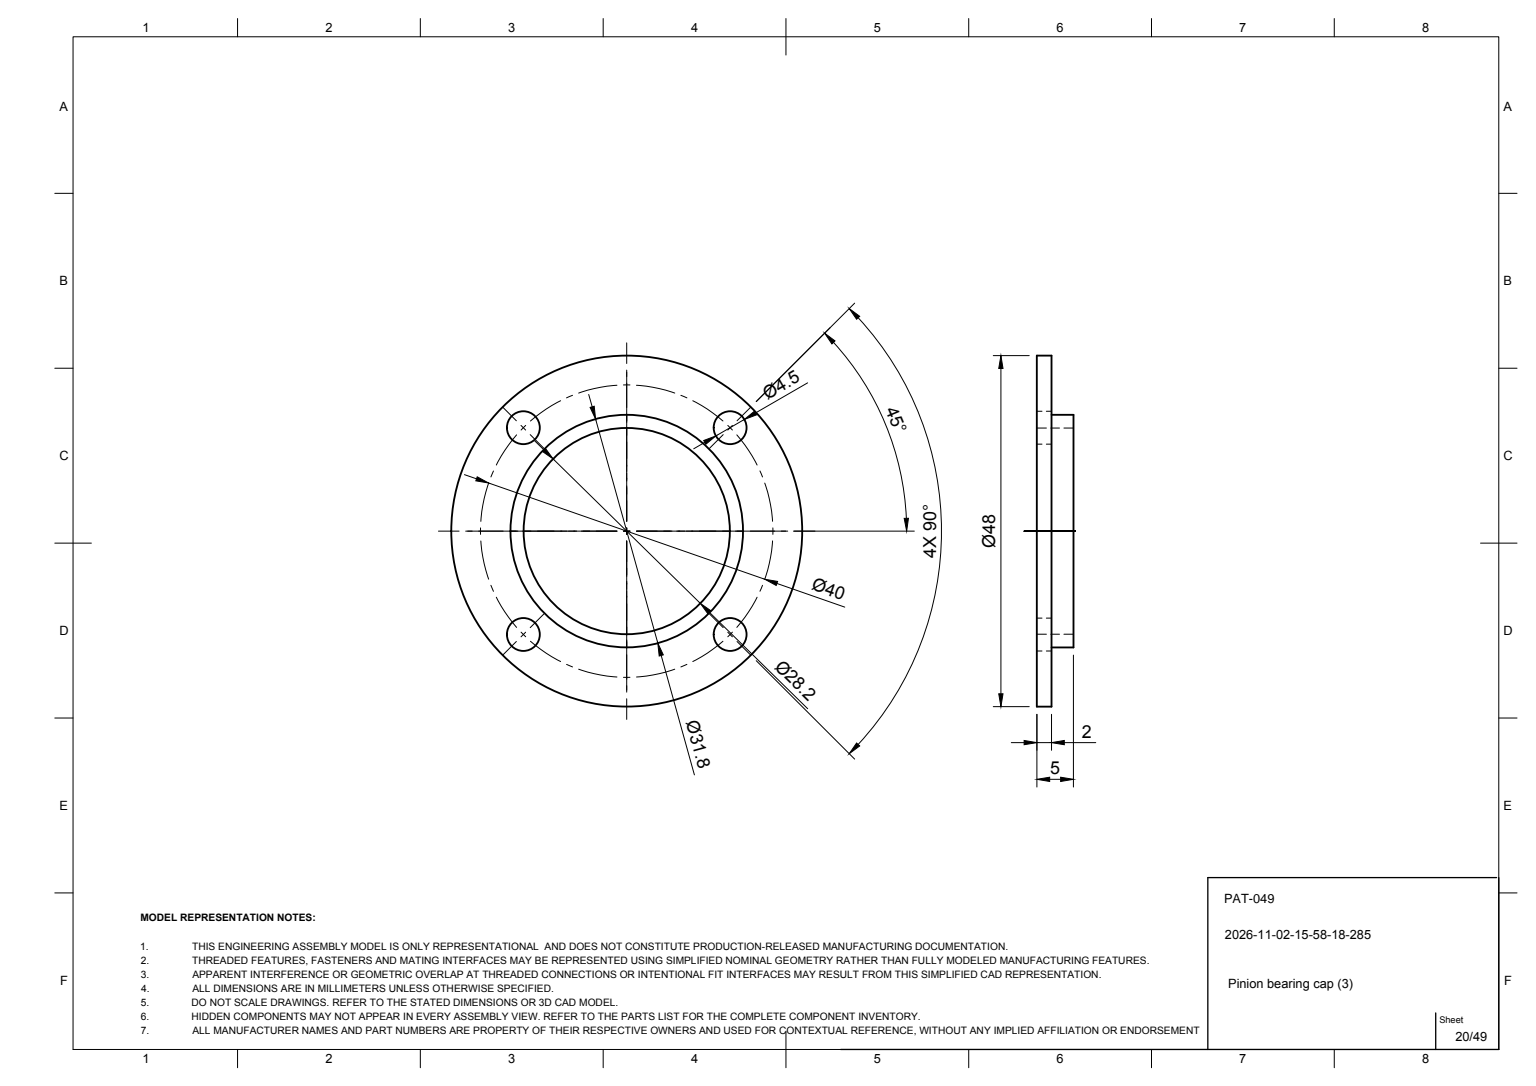
ISO-10303-21;
HEADER;
/* Generated by software containing ST-Developer
 * from STEP Tools, Inc. (www.steptools.com) 
 */

FILE_DESCRIPTION(
/* description */ ('Hand drill press frame (manual)'),
/* implementation_level */ '2;1');

FILE_NAME(
/* name */ 'Pinion bearing cap (3).step',
/* time_stamp */ '2026-10-28T03:25:28-07:00',
/* author */ (''),
/* organization */ (''),
/* preprocessor_version */ 'ST-DEVELOPER v20.2',
/* originating_system */ 'Autodesk Translation Framework v15.17.0.0',
/* authorisation */ '');

FILE_SCHEMA (('AUTOMOTIVE_DESIGN { 1 0 10303 214 3 1 1 }'));
ENDSEC;

DATA;
#10=MECHANICAL_DESIGN_GEOMETRIC_PRESENTATION_REPRESENTATION('',(#634),#33299);
#544=SHAPE_REPRESENTATION_RELATIONSHIP('SRR','None',#33503,#589);
#589=ADVANCED_BREP_SHAPE_REPRESENTATION('',(#686),#33265);
#634=STYLED_ITEM('',(#33814),#686);
#686=MANIFOLD_SOLID_BREP('Body1',#12652);
#825=FACE_BOUND('',#2342,.T.);
#826=FACE_BOUND('',#2346,.T.);
#827=FACE_BOUND('',#2347,.T.);
#828=FACE_BOUND('',#2348,.T.);
#829=FACE_BOUND('',#2349,.T.);
#830=FACE_BOUND('',#2350,.T.);
#831=FACE_BOUND('',#2352,.T.);
#832=FACE_BOUND('',#2353,.T.);
#833=FACE_BOUND('',#2354,.T.);
#834=FACE_BOUND('',#2355,.T.);
#835=FACE_BOUND('',#2356,.T.);
#1012=PLANE('',#13586);
#1013=PLANE('',#13593);
#1014=PLANE('',#13594);
#1542=FACE_OUTER_BOUND('',#2336,.T.);
#1543=FACE_OUTER_BOUND('',#2337,.T.);
#1544=FACE_OUTER_BOUND('',#2338,.T.);
#1545=FACE_OUTER_BOUND('',#2339,.T.);
#1546=FACE_OUTER_BOUND('',#2340,.T.);
#1547=FACE_OUTER_BOUND('',#2341,.T.);
#1548=FACE_OUTER_BOUND('',#2343,.T.);
#1549=FACE_OUTER_BOUND('',#2344,.T.);
#1550=FACE_OUTER_BOUND('',#2345,.T.);
#1551=FACE_OUTER_BOUND('',#2351,.T.);
#2336=EDGE_LOOP('',(#9395,#9396,#9397,#9398));
#2337=EDGE_LOOP('',(#9399,#9400,#9401,#9402));
#2338=EDGE_LOOP('',(#9403,#9404,#9405,#9406));
#2339=EDGE_LOOP('',(#9407,#9408,#9409,#9410));
#2340=EDGE_LOOP('',(#9411,#9412,#9413,#9414));
#2341=EDGE_LOOP('',(#9415));
#2342=EDGE_LOOP('',(#9416));
#2343=EDGE_LOOP('',(#9417,#9418,#9419,#9420));
#2344=EDGE_LOOP('',(#9421,#9422,#9423,#9424));
#2345=EDGE_LOOP('',(#9425));
#2346=EDGE_LOOP('',(#9426));
#2347=EDGE_LOOP('',(#9427));
#2348=EDGE_LOOP('',(#9428));
#2349=EDGE_LOOP('',(#9429));
#2350=EDGE_LOOP('',(#9430));
#2351=EDGE_LOOP('',(#9431));
#2352=EDGE_LOOP('',(#9432));
#2353=EDGE_LOOP('',(#9433));
#2354=EDGE_LOOP('',(#9434));
#2355=EDGE_LOOP('',(#9435));
#2356=EDGE_LOOP('',(#9436));
#3194=LINE('',#19110,#4359);
#3195=LINE('',#19116,#4360);
#3196=LINE('',#19122,#4361);
#3197=LINE('',#19128,#4362);
#3198=LINE('',#19134,#4363);
#3199=LINE('',#19142,#4364);
#3200=LINE('',#19147,#4365);
#4359=VECTOR('',#15447,0.225);
#4360=VECTOR('',#15454,0.225);
#4361=VECTOR('',#15461,0.225);
#4362=VECTOR('',#15468,0.225);
#4363=VECTOR('',#15475,1.59);
#4364=VECTOR('',#15486,1.41);
#4365=VECTOR('',#15491,2.4);
#5376=CIRCLE('',#13572,0.225);
#5377=CIRCLE('',#13573,0.225);
#5378=CIRCLE('',#13575,0.225);
#5379=CIRCLE('',#13576,0.225);
#5380=CIRCLE('',#13578,0.225);
#5381=CIRCLE('',#13579,0.225);
#5382=CIRCLE('',#13581,0.225);
#5383=CIRCLE('',#13582,0.225);
#5384=CIRCLE('',#13584,1.59);
#5385=CIRCLE('',#13585,1.59);
#5386=CIRCLE('',#13587,1.41);
#5387=CIRCLE('',#13589,1.41);
#5388=CIRCLE('',#13591,2.4);
#5389=CIRCLE('',#13592,2.4);
#5938=VERTEX_POINT('',#19107);
#5939=VERTEX_POINT('',#19109);
#5940=VERTEX_POINT('',#19113);
#5941=VERTEX_POINT('',#19115);
#5942=VERTEX_POINT('',#19119);
#5943=VERTEX_POINT('',#19121);
#5944=VERTEX_POINT('',#19125);
#5945=VERTEX_POINT('',#19127);
#5946=VERTEX_POINT('',#19131);
#5947=VERTEX_POINT('',#19133);
#5948=VERTEX_POINT('',#19137);
#5949=VERTEX_POINT('',#19140);
#5950=VERTEX_POINT('',#19144);
#5951=VERTEX_POINT('',#19146);
#7226=EDGE_CURVE('',#5938,#5938,#5376,.T.);
#7227=EDGE_CURVE('',#5938,#5939,#3194,.T.);
#7228=EDGE_CURVE('',#5939,#5939,#5377,.T.);
#7229=EDGE_CURVE('',#5940,#5940,#5378,.T.);
#7230=EDGE_CURVE('',#5940,#5941,#3195,.T.);
#7231=EDGE_CURVE('',#5941,#5941,#5379,.T.);
#7232=EDGE_CURVE('',#5942,#5942,#5380,.T.);
#7233=EDGE_CURVE('',#5942,#5943,#3196,.T.);
#7234=EDGE_CURVE('',#5943,#5943,#5381,.T.);
#7235=EDGE_CURVE('',#5944,#5944,#5382,.T.);
#7236=EDGE_CURVE('',#5944,#5945,#3197,.T.);
#7237=EDGE_CURVE('',#5945,#5945,#5383,.T.);
#7238=EDGE_CURVE('',#5946,#5946,#5384,.T.);
#7239=EDGE_CURVE('',#5946,#5947,#3198,.T.);
#7240=EDGE_CURVE('',#5947,#5947,#5385,.T.);
#7241=EDGE_CURVE('',#5948,#5948,#5386,.T.);
#7242=EDGE_CURVE('',#5949,#5949,#5387,.T.);
#7243=EDGE_CURVE('',#5949,#5948,#3199,.T.);
#7244=EDGE_CURVE('',#5950,#5950,#5388,.T.);
#7245=EDGE_CURVE('',#5950,#5951,#3200,.T.);
#7246=EDGE_CURVE('',#5951,#5951,#5389,.T.);
#9395=ORIENTED_EDGE('',*,*,#7226,.F.);
#9396=ORIENTED_EDGE('',*,*,#7227,.T.);
#9397=ORIENTED_EDGE('',*,*,#7228,.F.);
#9398=ORIENTED_EDGE('',*,*,#7227,.F.);
#9399=ORIENTED_EDGE('',*,*,#7229,.F.);
#9400=ORIENTED_EDGE('',*,*,#7230,.T.);
#9401=ORIENTED_EDGE('',*,*,#7231,.F.);
#9402=ORIENTED_EDGE('',*,*,#7230,.F.);
#9403=ORIENTED_EDGE('',*,*,#7232,.F.);
#9404=ORIENTED_EDGE('',*,*,#7233,.T.);
#9405=ORIENTED_EDGE('',*,*,#7234,.F.);
#9406=ORIENTED_EDGE('',*,*,#7233,.F.);
#9407=ORIENTED_EDGE('',*,*,#7235,.F.);
#9408=ORIENTED_EDGE('',*,*,#7236,.T.);
#9409=ORIENTED_EDGE('',*,*,#7237,.F.);
#9410=ORIENTED_EDGE('',*,*,#7236,.F.);
#9411=ORIENTED_EDGE('',*,*,#7238,.F.);
#9412=ORIENTED_EDGE('',*,*,#7239,.T.);
#9413=ORIENTED_EDGE('',*,*,#7240,.T.);
#9414=ORIENTED_EDGE('',*,*,#7239,.F.);
#9415=ORIENTED_EDGE('',*,*,#7240,.F.);
#9416=ORIENTED_EDGE('',*,*,#7241,.F.);
#9417=ORIENTED_EDGE('',*,*,#7242,.F.);
#9418=ORIENTED_EDGE('',*,*,#7243,.T.);
#9419=ORIENTED_EDGE('',*,*,#7241,.T.);
#9420=ORIENTED_EDGE('',*,*,#7243,.F.);
#9421=ORIENTED_EDGE('',*,*,#7244,.F.);
#9422=ORIENTED_EDGE('',*,*,#7245,.T.);
#9423=ORIENTED_EDGE('',*,*,#7246,.T.);
#9424=ORIENTED_EDGE('',*,*,#7245,.F.);
#9425=ORIENTED_EDGE('',*,*,#7244,.T.);
#9426=ORIENTED_EDGE('',*,*,#7242,.T.);
#9427=ORIENTED_EDGE('',*,*,#7237,.T.);
#9428=ORIENTED_EDGE('',*,*,#7234,.T.);
#9429=ORIENTED_EDGE('',*,*,#7231,.T.);
#9430=ORIENTED_EDGE('',*,*,#7228,.T.);
#9431=ORIENTED_EDGE('',*,*,#7246,.F.);
#9432=ORIENTED_EDGE('',*,*,#7238,.T.);
#9433=ORIENTED_EDGE('',*,*,#7235,.T.);
#9434=ORIENTED_EDGE('',*,*,#7232,.T.);
#9435=ORIENTED_EDGE('',*,*,#7229,.T.);
#9436=ORIENTED_EDGE('',*,*,#7226,.T.);
#11863=CYLINDRICAL_SURFACE('',#13571,0.225);
#11864=CYLINDRICAL_SURFACE('',#13574,0.225);
#11865=CYLINDRICAL_SURFACE('',#13577,0.225);
#11866=CYLINDRICAL_SURFACE('',#13580,0.225);
#11867=CYLINDRICAL_SURFACE('',#13583,1.59);
#11868=CYLINDRICAL_SURFACE('',#13588,1.41);
#11869=CYLINDRICAL_SURFACE('',#13590,2.4);
#12151=ADVANCED_FACE('',(#1542),#11863,.F.);
#12152=ADVANCED_FACE('',(#1543),#11864,.F.);
#12153=ADVANCED_FACE('',(#1544),#11865,.F.);
#12154=ADVANCED_FACE('',(#1545),#11866,.F.);
#12155=ADVANCED_FACE('',(#1546),#11867,.T.);
#12156=ADVANCED_FACE('',(#1547,#825),#1012,.F.);
#12157=ADVANCED_FACE('',(#1548),#11868,.F.);
#12158=ADVANCED_FACE('',(#1549),#11869,.T.);
#12159=ADVANCED_FACE('',(#1550,#826,#827,#828,#829,#830),#1013,.T.);
#12160=ADVANCED_FACE('',(#1551,#831,#832,#833,#834,#835),#1014,.F.);
#12652=CLOSED_SHELL('',(#12151,#12152,#12153,#12154,#12155,#12156,#12157,
#12158,#12159,#12160));
#13570=AXIS2_PLACEMENT_3D('',#19105,#15441,#15442);
#13571=AXIS2_PLACEMENT_3D('',#19106,#15443,#15444);
#13572=AXIS2_PLACEMENT_3D('',#19108,#15445,#15446);
#13573=AXIS2_PLACEMENT_3D('',#19111,#15448,#15449);
#13574=AXIS2_PLACEMENT_3D('',#19112,#15450,#15451);
#13575=AXIS2_PLACEMENT_3D('',#19114,#15452,#15453);
#13576=AXIS2_PLACEMENT_3D('',#19117,#15455,#15456);
#13577=AXIS2_PLACEMENT_3D('',#19118,#15457,#15458);
#13578=AXIS2_PLACEMENT_3D('',#19120,#15459,#15460);
#13579=AXIS2_PLACEMENT_3D('',#19123,#15462,#15463);
#13580=AXIS2_PLACEMENT_3D('',#19124,#15464,#15465);
#13581=AXIS2_PLACEMENT_3D('',#19126,#15466,#15467);
#13582=AXIS2_PLACEMENT_3D('',#19129,#15469,#15470);
#13583=AXIS2_PLACEMENT_3D('',#19130,#15471,#15472);
#13584=AXIS2_PLACEMENT_3D('',#19132,#15473,#15474);
#13585=AXIS2_PLACEMENT_3D('',#19135,#15476,#15477);
#13586=AXIS2_PLACEMENT_3D('',#19136,#15478,#15479);
#13587=AXIS2_PLACEMENT_3D('',#19138,#15480,#15481);
#13588=AXIS2_PLACEMENT_3D('',#19139,#15482,#15483);
#13589=AXIS2_PLACEMENT_3D('',#19141,#15484,#15485);
#13590=AXIS2_PLACEMENT_3D('',#19143,#15487,#15488);
#13591=AXIS2_PLACEMENT_3D('',#19145,#15489,#15490);
#13592=AXIS2_PLACEMENT_3D('',#19148,#15492,#15493);
#13593=AXIS2_PLACEMENT_3D('',#19149,#15494,#15495);
#13594=AXIS2_PLACEMENT_3D('',#19150,#15496,#15497);
#15441=DIRECTION('axis',(0.,0.,1.));
#15442=DIRECTION('refdir',(1.,0.,0.));
#15443=DIRECTION('center_axis',(0.,1.,0.));
#15444=DIRECTION('ref_axis',(1.,0.,0.));
#15445=DIRECTION('center_axis',(0.,1.,0.));
#15446=DIRECTION('ref_axis',(1.,0.,0.));
#15447=DIRECTION('',(0.,1.,0.));
#15448=DIRECTION('center_axis',(0.,-1.,0.));
#15449=DIRECTION('ref_axis',(1.,0.,0.));
#15450=DIRECTION('center_axis',(0.,1.,0.));
#15451=DIRECTION('ref_axis',(1.,0.,0.));
#15452=DIRECTION('center_axis',(0.,1.,0.));
#15453=DIRECTION('ref_axis',(1.,0.,0.));
#15454=DIRECTION('',(0.,1.,0.));
#15455=DIRECTION('center_axis',(0.,-1.,0.));
#15456=DIRECTION('ref_axis',(1.,0.,0.));
#15457=DIRECTION('center_axis',(0.,1.,0.));
#15458=DIRECTION('ref_axis',(1.,0.,0.));
#15459=DIRECTION('center_axis',(0.,1.,0.));
#15460=DIRECTION('ref_axis',(1.,0.,0.));
#15461=DIRECTION('',(0.,1.,0.));
#15462=DIRECTION('center_axis',(0.,-1.,0.));
#15463=DIRECTION('ref_axis',(1.,0.,0.));
#15464=DIRECTION('center_axis',(0.,1.,0.));
#15465=DIRECTION('ref_axis',(1.,0.,0.));
#15466=DIRECTION('center_axis',(0.,1.,0.));
#15467=DIRECTION('ref_axis',(1.,0.,0.));
#15468=DIRECTION('',(0.,1.,0.));
#15469=DIRECTION('center_axis',(0.,-1.,0.));
#15470=DIRECTION('ref_axis',(1.,0.,0.));
#15471=DIRECTION('center_axis',(0.,1.,0.));
#15472=DIRECTION('ref_axis',(1.,0.,0.));
#15473=DIRECTION('center_axis',(0.,1.,0.));
#15474=DIRECTION('ref_axis',(1.,0.,0.));
#15475=DIRECTION('',(0.,-1.,0.));
#15476=DIRECTION('center_axis',(0.,1.,0.));
#15477=DIRECTION('ref_axis',(1.,0.,0.));
#15478=DIRECTION('center_axis',(0.,1.,0.));
#15479=DIRECTION('ref_axis',(1.,0.,0.));
#15480=DIRECTION('center_axis',(0.,-1.,0.));
#15481=DIRECTION('ref_axis',(1.,0.,0.));
#15482=DIRECTION('center_axis',(0.,1.,0.));
#15483=DIRECTION('ref_axis',(1.,0.,0.));
#15484=DIRECTION('center_axis',(0.,-1.,0.));
#15485=DIRECTION('ref_axis',(1.,0.,0.));
#15486=DIRECTION('',(0.,-1.,0.));
#15487=DIRECTION('center_axis',(0.,1.,0.));
#15488=DIRECTION('ref_axis',(1.,0.,0.));
#15489=DIRECTION('center_axis',(0.,1.,0.));
#15490=DIRECTION('ref_axis',(1.,0.,0.));
#15491=DIRECTION('',(0.,-1.,0.));
#15492=DIRECTION('center_axis',(0.,1.,0.));
#15493=DIRECTION('ref_axis',(1.,0.,0.));
#15494=DIRECTION('center_axis',(0.,1.,0.));
#15495=DIRECTION('ref_axis',(1.,0.,0.));
#15496=DIRECTION('center_axis',(0.,1.,0.));
#15497=DIRECTION('ref_axis',(1.,0.,0.));
#19105=CARTESIAN_POINT('',(0.,0.,0.));
#19106=CARTESIAN_POINT('Origin',(-4.66421356237309,3.7,18.5857864376269));
#19107=CARTESIAN_POINT('',(-4.88921356237309,3.8,18.5857864376269));
#19108=CARTESIAN_POINT('Origin',(-4.66421356237309,3.8,18.5857864376269));
#19109=CARTESIAN_POINT('',(-4.88921356237309,4.,18.5857864376269));
#19110=CARTESIAN_POINT('',(-4.88921356237309,3.7,18.5857864376269));
#19111=CARTESIAN_POINT('Origin',(-4.66421356237309,4.,18.5857864376269));
#19112=CARTESIAN_POINT('Origin',(-4.66421356237309,3.7,21.4142135623731));
#19113=CARTESIAN_POINT('',(-4.88921356237309,3.8,21.4142135623731));
#19114=CARTESIAN_POINT('Origin',(-4.66421356237309,3.8,21.4142135623731));
#19115=CARTESIAN_POINT('',(-4.88921356237309,4.,21.4142135623731));
#19116=CARTESIAN_POINT('',(-4.88921356237309,3.7,21.4142135623731));
#19117=CARTESIAN_POINT('Origin',(-4.66421356237309,4.,21.4142135623731));
#19118=CARTESIAN_POINT('Origin',(-1.8357864376269,3.7,21.4142135623731));
#19119=CARTESIAN_POINT('',(-2.0607864376269,3.8,21.4142135623731));
#19120=CARTESIAN_POINT('Origin',(-1.8357864376269,3.8,21.4142135623731));
#19121=CARTESIAN_POINT('',(-2.0607864376269,4.,21.4142135623731));
#19122=CARTESIAN_POINT('',(-2.0607864376269,3.7,21.4142135623731));
#19123=CARTESIAN_POINT('Origin',(-1.8357864376269,4.,21.4142135623731));
#19124=CARTESIAN_POINT('Origin',(-1.83578643762691,3.7,18.5857864376269));
#19125=CARTESIAN_POINT('',(-2.06078643762691,3.8,18.5857864376269));
#19126=CARTESIAN_POINT('Origin',(-1.83578643762691,3.8,18.5857864376269));
#19127=CARTESIAN_POINT('',(-2.06078643762691,4.,18.5857864376269));
#19128=CARTESIAN_POINT('',(-2.06078643762691,3.7,18.5857864376269));
#19129=CARTESIAN_POINT('Origin',(-1.83578643762691,4.,18.5857864376269));
#19130=CARTESIAN_POINT('Origin',(-3.25,3.5,20.));
#19131=CARTESIAN_POINT('',(-4.84,3.8,20.));
#19132=CARTESIAN_POINT('Origin',(-3.25,3.8,20.));
#19133=CARTESIAN_POINT('',(-4.84,3.5,20.));
#19134=CARTESIAN_POINT('',(-4.84,3.5,20.));
#19135=CARTESIAN_POINT('Origin',(-3.25,3.5,20.));
#19136=CARTESIAN_POINT('Origin',(-3.25,3.5,20.));
#19137=CARTESIAN_POINT('',(-4.66,3.5,20.));
#19138=CARTESIAN_POINT('Origin',(-3.25,3.5,20.));
#19139=CARTESIAN_POINT('Origin',(-3.25,3.8,20.));
#19140=CARTESIAN_POINT('',(-4.66,4.,20.));
#19141=CARTESIAN_POINT('Origin',(-3.25,4.,20.));
#19142=CARTESIAN_POINT('',(-4.66,3.8,20.));
#19143=CARTESIAN_POINT('Origin',(-3.25,3.8,20.));
#19144=CARTESIAN_POINT('',(-5.65,4.,20.));
#19145=CARTESIAN_POINT('Origin',(-3.25,4.,20.));
#19146=CARTESIAN_POINT('',(-5.65,3.8,20.));
#19147=CARTESIAN_POINT('',(-5.65,3.8,20.));
#19148=CARTESIAN_POINT('Origin',(-3.25,3.8,20.));
#19149=CARTESIAN_POINT('Origin',(-3.25,4.,20.));
#19150=CARTESIAN_POINT('Origin',(-3.25,3.8,20.));
#33213=UNCERTAINTY_MEASURE_WITH_UNIT(LENGTH_MEASURE(0.001),#33300,
'DISTANCE_ACCURACY_VALUE',
'Maximum model space distance between geometric entities at asserted c
onnectivities');
#33247=UNCERTAINTY_MEASURE_WITH_UNIT(LENGTH_MEASURE(0.001),#33300,
'DISTANCE_ACCURACY_VALUE',
'Maximum model space distance between geometric entities at asserted c
onnectivities');
#33265=(
GEOMETRIC_REPRESENTATION_CONTEXT(3)
GLOBAL_UNCERTAINTY_ASSIGNED_CONTEXT((#33213))
GLOBAL_UNIT_ASSIGNED_CONTEXT((#33300,#33302,#33303))
REPRESENTATION_CONTEXT('','3D')
);
#33299=(
GEOMETRIC_REPRESENTATION_CONTEXT(3)
GLOBAL_UNCERTAINTY_ASSIGNED_CONTEXT((#33247))
GLOBAL_UNIT_ASSIGNED_CONTEXT((#33300,#33302,#33303))
REPRESENTATION_CONTEXT('','3D')
);
#33300=(
LENGTH_UNIT()
NAMED_UNIT(*)
SI_UNIT(.CENTI.,.METRE.)
);
#33302=(
NAMED_UNIT(*)
PLANE_ANGLE_UNIT()
SI_UNIT($,.RADIAN.)
);
#33303=(
NAMED_UNIT(*)
SI_UNIT($,.STERADIAN.)
SOLID_ANGLE_UNIT()
);
#33321=SHAPE_DEFINITION_REPRESENTATION(#33372,#33503);
#33372=PRODUCT_DEFINITION_SHAPE('',$,#33555);
#33503=SHAPE_REPRESENTATION('',(#13570),#33265);
#33537=PRODUCT_DEFINITION_CONTEXT('part definition',#33692,'design');
#33555=PRODUCT_DEFINITION('Pinion bearing cap (3)',
'Pinion bearing cap (3)',#33606,#33537);
#33606=PRODUCT_DEFINITION_FORMATION('',$,#33711);
#33692=APPLICATION_CONTEXT(
'Core Data for Automotive Mechanical Design Process');
#33693=PRODUCT_CONTEXT('part definition',#33692,'mechanical');
#33711=PRODUCT('Pinion bearing cap (3)','Pinion bearing cap (3)',
'Pinion bearing cap (3)',(#33693));
#33808=COLOUR_RGB('Grey',0.48,0.52,0.57);
#33809=FILL_AREA_STYLE_COLOUR('',#33808);
#33810=FILL_AREA_STYLE('',(#33809));
#33811=SURFACE_STYLE_FILL_AREA(#33810);
#33812=SURFACE_SIDE_STYLE('',(#33811));
#33813=SURFACE_STYLE_USAGE(.BOTH.,#33812);
#33814=PRESENTATION_STYLE_ASSIGNMENT((#33813));
ENDSEC;
END-ISO-10303-21;
